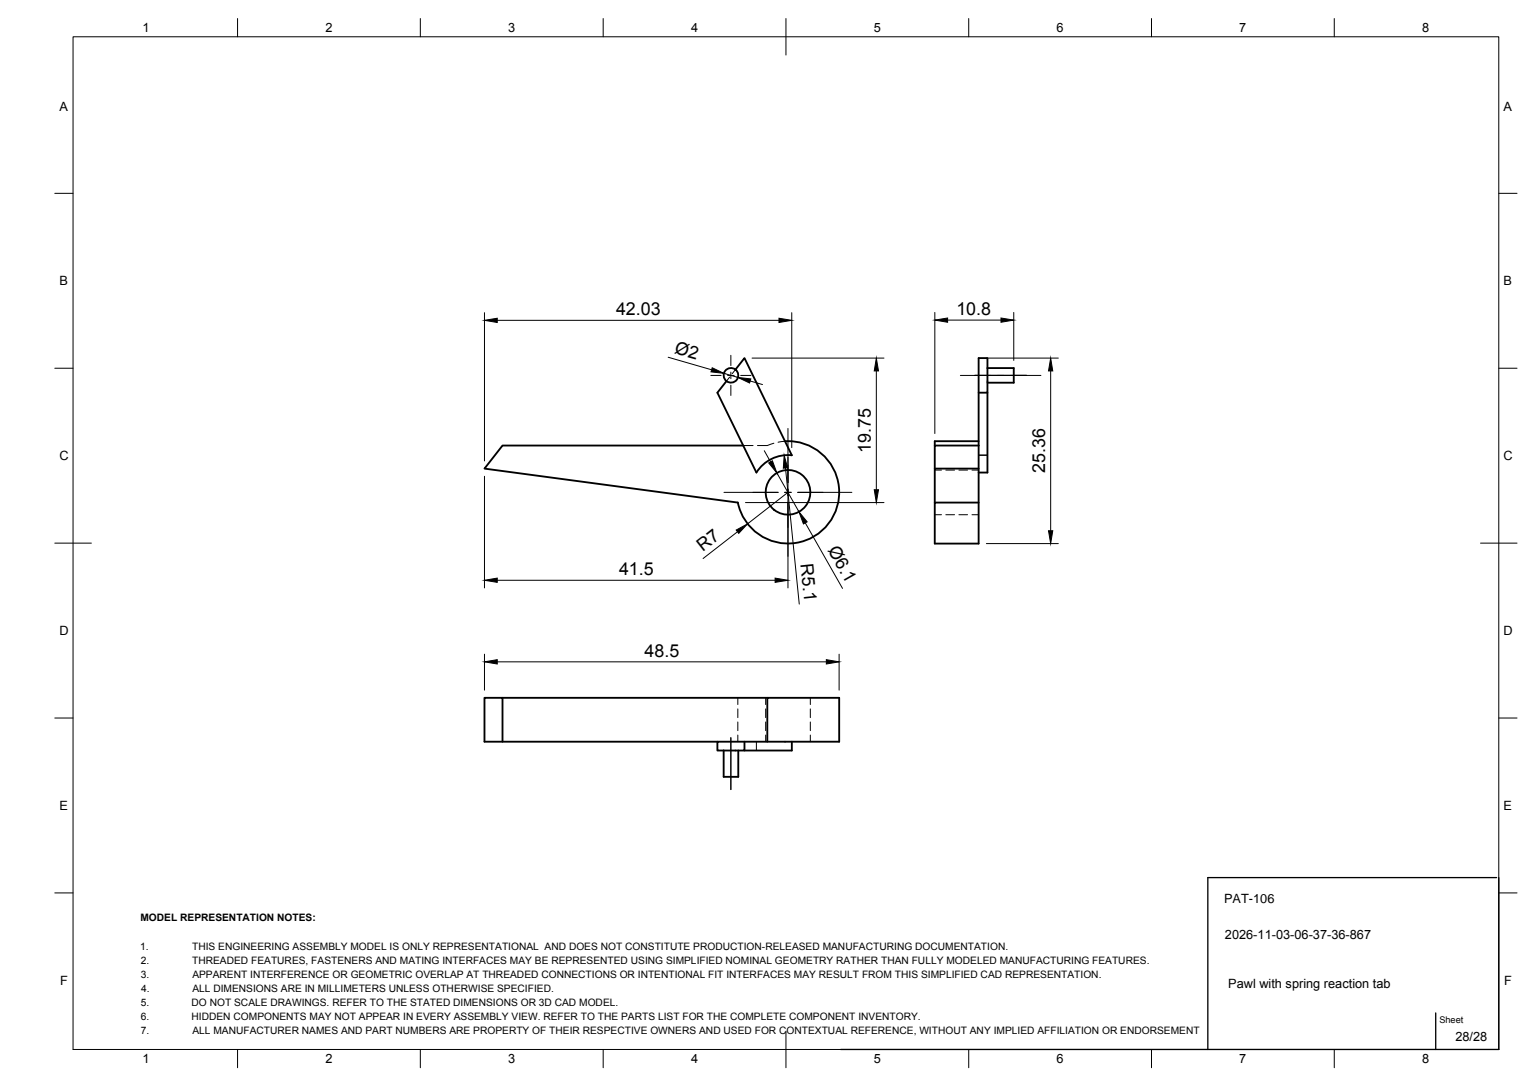
ISO-10303-21;
HEADER;
/* Generated by software containing ST-Developer
 * from STEP Tools, Inc. (www.steptools.com) 
 */

FILE_DESCRIPTION(
/* description */ ('Torsion-spring ratchet demonstrator'),
/* implementation_level */ '2;1');

FILE_NAME(
/* name */ 'Pawl with spring reaction tab.step',
/* time_stamp */ '2026-10-29T17:29:17-07:00',
/* author */ (''),
/* organization */ (''),
/* preprocessor_version */ 'ST-DEVELOPER v20.2',
/* originating_system */ 'Autodesk Translation Framework v15.17.0.0',
/* authorisation */ '');

FILE_SCHEMA (('AUTOMOTIVE_DESIGN { 1 0 10303 214 3 1 1 }'));
ENDSEC;

DATA;
#10=MECHANICAL_DESIGN_GEOMETRIC_PRESENTATION_REPRESENTATION('',(#314),#11258);
#258=SHAPE_REPRESENTATION_RELATIONSHIP('SRR','None',#11387,#282);
#282=ADVANCED_BREP_SHAPE_REPRESENTATION('',(#344),#11257);
#314=STYLED_ITEM('',(#11584),#344);
#344=MANIFOLD_SOLID_BREP('Body1',#5187);
#435=FACE_BOUND('',#1309,.T.);
#436=FACE_BOUND('',#1324,.T.);
#611=PLANE('',#6039);
#612=PLANE('',#6046);
#613=PLANE('',#6047);
#614=PLANE('',#6048);
#615=PLANE('',#6050);
#616=PLANE('',#6051);
#617=PLANE('',#6052);
#618=PLANE('',#6053);
#619=PLANE('',#6058);
#620=PLANE('',#6059);
#621=PLANE('',#6060);
#622=PLANE('',#6061);
#912=FACE_OUTER_BOUND('',#1307,.T.);
#913=FACE_OUTER_BOUND('',#1308,.T.);
#914=FACE_OUTER_BOUND('',#1310,.T.);
#915=FACE_OUTER_BOUND('',#1311,.T.);
#916=FACE_OUTER_BOUND('',#1312,.T.);
#917=FACE_OUTER_BOUND('',#1313,.T.);
#918=FACE_OUTER_BOUND('',#1314,.T.);
#919=FACE_OUTER_BOUND('',#1315,.T.);
#920=FACE_OUTER_BOUND('',#1316,.T.);
#921=FACE_OUTER_BOUND('',#1317,.T.);
#922=FACE_OUTER_BOUND('',#1318,.T.);
#923=FACE_OUTER_BOUND('',#1319,.T.);
#924=FACE_OUTER_BOUND('',#1320,.T.);
#925=FACE_OUTER_BOUND('',#1321,.T.);
#926=FACE_OUTER_BOUND('',#1322,.T.);
#927=FACE_OUTER_BOUND('',#1323,.T.);
#1307=EDGE_LOOP('',(#4690,#4691,#4692,#4693));
#1308=EDGE_LOOP('',(#4694,#4695,#4696,#4697,#4698,#4699,#4700));
#1309=EDGE_LOOP('',(#4701));
#1310=EDGE_LOOP('',(#4702,#4703,#4704,#4705,#4706));
#1311=EDGE_LOOP('',(#4707));
#1312=EDGE_LOOP('',(#4708,#4709));
#1313=EDGE_LOOP('',(#4710,#4711,#4712,#4713,#4714));
#1314=EDGE_LOOP('',(#4715,#4716,#4717,#4718,#4719,#4720));
#1315=EDGE_LOOP('',(#4721,#4722,#4723,#4724,#4725));
#1316=EDGE_LOOP('',(#4726,#4727,#4728,#4729,#4730));
#1317=EDGE_LOOP('',(#4731,#4732,#4733,#4734,#4735,#4736));
#1318=EDGE_LOOP('',(#4737,#4738,#4739,#4740));
#1319=EDGE_LOOP('',(#4741,#4742,#4743,#4744,#4745));
#1320=EDGE_LOOP('',(#4746,#4747,#4748,#4749));
#1321=EDGE_LOOP('',(#4750,#4751,#4752,#4753));
#1322=EDGE_LOOP('',(#4754,#4755,#4756,#4757,#4758));
#1323=EDGE_LOOP('',(#4759,#4760,#4761,#4762));
#1324=EDGE_LOOP('',(#4763));
#1681=LINE('',#11122,#2064);
#1682=LINE('',#11126,#2065);
#1683=LINE('',#11130,#2066);
#1684=LINE('',#11132,#2067);
#1685=LINE('',#11134,#2068);
#1686=LINE('',#11136,#2069);
#1687=LINE('',#11139,#2070);
#1688=LINE('',#11146,#2071);
#1689=LINE('',#11152,#2072);
#1690=LINE('',#11156,#2073);
#1691=LINE('',#11158,#2074);
#1692=LINE('',#11160,#2075);
#1693=LINE('',#11161,#2076);
#1694=LINE('',#11164,#2077);
#1695=LINE('',#11165,#2078);
#1696=LINE('',#11167,#2079);
#1697=LINE('',#11168,#2080);
#1698=LINE('',#11170,#2081);
#1699=LINE('',#11172,#2082);
#1700=LINE('',#11177,#2083);
#1701=LINE('',#11180,#2084);
#1702=LINE('',#11183,#2085);
#1703=LINE('',#11186,#2086);
#1704=LINE('',#11187,#2087);
#1705=LINE('',#11190,#2088);
#1706=LINE('',#11191,#2089);
#1707=LINE('',#11193,#2090);
#2064=VECTOR('',#7590,1.);
#2065=VECTOR('',#7593,1.);
#2066=VECTOR('',#7598,1.);
#2067=VECTOR('',#7599,1.);
#2068=VECTOR('',#7600,1.);
#2069=VECTOR('',#7601,1.);
#2070=VECTOR('',#7604,1.);
#2071=VECTOR('',#7611,0.0999999999999996);
#2072=VECTOR('',#7620,1.);
#2073=VECTOR('',#7625,1.);
#2074=VECTOR('',#7626,1.);
#2075=VECTOR('',#7627,1.);
#2076=VECTOR('',#7628,1.);
#2077=VECTOR('',#7631,1.);
#2078=VECTOR('',#7632,1.);
#2079=VECTOR('',#7633,1.);
#2080=VECTOR('',#7634,1.);
#2081=VECTOR('',#7637,1.);
#2082=VECTOR('',#7640,1.);
#2083=VECTOR('',#7647,0.305);
#2084=VECTOR('',#7650,1.);
#2085=VECTOR('',#7653,1.);
#2086=VECTOR('',#7656,1.);
#2087=VECTOR('',#7657,1.);
#2088=VECTOR('',#7660,1.);
#2089=VECTOR('',#7661,1.);
#2090=VECTOR('',#7664,1.);
#2325=CIRCLE('',#6037,0.51);
#2326=CIRCLE('',#6038,0.51);
#2327=CIRCLE('',#6040,0.7);
#2328=CIRCLE('',#6041,0.305);
#2329=CIRCLE('',#6043,0.0999999999999996);
#2330=CIRCLE('',#6044,0.0999999999999996);
#2331=CIRCLE('',#6045,0.0999999999999996);
#2332=CIRCLE('',#6049,0.7);
#2333=CIRCLE('',#6055,0.305);
#2334=CIRCLE('',#6057,0.7);
#2758=VERTEX_POINT('',#11120);
#2759=VERTEX_POINT('',#11121);
#2760=VERTEX_POINT('',#11123);
#2761=VERTEX_POINT('',#11125);
#2762=VERTEX_POINT('',#11129);
#2763=VERTEX_POINT('',#11131);
#2764=VERTEX_POINT('',#11133);
#2765=VERTEX_POINT('',#11135);
#2766=VERTEX_POINT('',#11137);
#2767=VERTEX_POINT('',#11140);
#2768=VERTEX_POINT('',#11143);
#2769=VERTEX_POINT('',#11145);
#2770=VERTEX_POINT('',#11147);
#2771=VERTEX_POINT('',#11154);
#2772=VERTEX_POINT('',#11157);
#2773=VERTEX_POINT('',#11159);
#2774=VERTEX_POINT('',#11163);
#2775=VERTEX_POINT('',#11166);
#2776=VERTEX_POINT('',#11175);
#2777=VERTEX_POINT('',#11179);
#2778=VERTEX_POINT('',#11181);
#2779=VERTEX_POINT('',#11185);
#2780=VERTEX_POINT('',#11189);
#3405=EDGE_CURVE('',#2758,#2759,#1681,.T.);
#3406=EDGE_CURVE('',#2760,#2758,#2325,.T.);
#3407=EDGE_CURVE('',#2761,#2760,#1682,.T.);
#3408=EDGE_CURVE('',#2759,#2761,#2326,.T.);
#3409=EDGE_CURVE('',#2761,#2762,#1683,.T.);
#3410=EDGE_CURVE('',#2762,#2763,#1684,.T.);
#3411=EDGE_CURVE('',#2763,#2764,#1685,.T.);
#3412=EDGE_CURVE('',#2764,#2765,#1686,.T.);
#3413=EDGE_CURVE('',#2765,#2766,#2327,.T.);
#3414=EDGE_CURVE('',#2766,#2759,#1687,.T.);
#3415=EDGE_CURVE('',#2767,#2767,#2328,.T.);
#3416=EDGE_CURVE('',#2768,#2768,#2329,.T.);
#3417=EDGE_CURVE('',#2768,#2769,#1688,.T.);
#3418=EDGE_CURVE('',#2770,#2769,#2330,.T.);
#3419=EDGE_CURVE('',#2770,#2769,#2331,.T.);
#3420=EDGE_CURVE('',#2770,#2769,#1689,.T.);
#3421=EDGE_CURVE('',#2766,#2771,#2332,.T.);
#3422=EDGE_CURVE('',#2771,#2762,#1690,.T.);
#3423=EDGE_CURVE('',#2772,#2762,#1691,.T.);
#3424=EDGE_CURVE('',#2773,#2772,#1692,.T.);
#3425=EDGE_CURVE('',#2766,#2773,#1693,.T.);
#3426=EDGE_CURVE('',#2772,#2774,#1694,.T.);
#3427=EDGE_CURVE('',#2769,#2774,#1695,.T.);
#3428=EDGE_CURVE('',#2775,#2770,#1696,.T.);
#3429=EDGE_CURVE('',#2773,#2775,#1697,.T.);
#3430=EDGE_CURVE('',#2758,#2775,#1698,.T.);
#3431=EDGE_CURVE('',#2774,#2760,#1699,.T.);
#3432=EDGE_CURVE('',#2776,#2776,#2333,.T.);
#3433=EDGE_CURVE('',#2776,#2767,#1700,.T.);
#3434=EDGE_CURVE('',#2777,#2765,#1701,.T.);
#3435=EDGE_CURVE('',#2777,#2778,#2334,.T.);
#3436=EDGE_CURVE('',#2771,#2778,#1702,.T.);
#3437=EDGE_CURVE('',#2779,#2764,#1703,.T.);
#3438=EDGE_CURVE('',#2777,#2779,#1704,.T.);
#3439=EDGE_CURVE('',#2779,#2780,#1705,.T.);
#3440=EDGE_CURVE('',#2780,#2763,#1706,.T.);
#3441=EDGE_CURVE('',#2780,#2778,#1707,.T.);
#4690=ORIENTED_EDGE('',*,*,#3405,.F.);
#4691=ORIENTED_EDGE('',*,*,#3406,.F.);
#4692=ORIENTED_EDGE('',*,*,#3407,.F.);
#4693=ORIENTED_EDGE('',*,*,#3408,.F.);
#4694=ORIENTED_EDGE('',*,*,#3408,.T.);
#4695=ORIENTED_EDGE('',*,*,#3409,.T.);
#4696=ORIENTED_EDGE('',*,*,#3410,.T.);
#4697=ORIENTED_EDGE('',*,*,#3411,.T.);
#4698=ORIENTED_EDGE('',*,*,#3412,.T.);
#4699=ORIENTED_EDGE('',*,*,#3413,.T.);
#4700=ORIENTED_EDGE('',*,*,#3414,.T.);
#4701=ORIENTED_EDGE('',*,*,#3415,.T.);
#4702=ORIENTED_EDGE('',*,*,#3416,.F.);
#4703=ORIENTED_EDGE('',*,*,#3417,.T.);
#4704=ORIENTED_EDGE('',*,*,#3418,.F.);
#4705=ORIENTED_EDGE('',*,*,#3419,.T.);
#4706=ORIENTED_EDGE('',*,*,#3417,.F.);
#4707=ORIENTED_EDGE('',*,*,#3416,.T.);
#4708=ORIENTED_EDGE('',*,*,#3420,.T.);
#4709=ORIENTED_EDGE('',*,*,#3419,.F.);
#4710=ORIENTED_EDGE('',*,*,#3421,.T.);
#4711=ORIENTED_EDGE('',*,*,#3422,.T.);
#4712=ORIENTED_EDGE('',*,*,#3423,.F.);
#4713=ORIENTED_EDGE('',*,*,#3424,.F.);
#4714=ORIENTED_EDGE('',*,*,#3425,.F.);
#4715=ORIENTED_EDGE('',*,*,#3424,.T.);
#4716=ORIENTED_EDGE('',*,*,#3426,.T.);
#4717=ORIENTED_EDGE('',*,*,#3427,.F.);
#4718=ORIENTED_EDGE('',*,*,#3420,.F.);
#4719=ORIENTED_EDGE('',*,*,#3428,.F.);
#4720=ORIENTED_EDGE('',*,*,#3429,.F.);
#4721=ORIENTED_EDGE('',*,*,#3405,.T.);
#4722=ORIENTED_EDGE('',*,*,#3414,.F.);
#4723=ORIENTED_EDGE('',*,*,#3425,.T.);
#4724=ORIENTED_EDGE('',*,*,#3429,.T.);
#4725=ORIENTED_EDGE('',*,*,#3430,.F.);
#4726=ORIENTED_EDGE('',*,*,#3407,.T.);
#4727=ORIENTED_EDGE('',*,*,#3431,.F.);
#4728=ORIENTED_EDGE('',*,*,#3426,.F.);
#4729=ORIENTED_EDGE('',*,*,#3423,.T.);
#4730=ORIENTED_EDGE('',*,*,#3409,.F.);
#4731=ORIENTED_EDGE('',*,*,#3406,.T.);
#4732=ORIENTED_EDGE('',*,*,#3430,.T.);
#4733=ORIENTED_EDGE('',*,*,#3428,.T.);
#4734=ORIENTED_EDGE('',*,*,#3418,.T.);
#4735=ORIENTED_EDGE('',*,*,#3427,.T.);
#4736=ORIENTED_EDGE('',*,*,#3431,.T.);
#4737=ORIENTED_EDGE('',*,*,#3432,.F.);
#4738=ORIENTED_EDGE('',*,*,#3433,.T.);
#4739=ORIENTED_EDGE('',*,*,#3415,.F.);
#4740=ORIENTED_EDGE('',*,*,#3433,.F.);
#4741=ORIENTED_EDGE('',*,*,#3434,.F.);
#4742=ORIENTED_EDGE('',*,*,#3435,.T.);
#4743=ORIENTED_EDGE('',*,*,#3436,.F.);
#4744=ORIENTED_EDGE('',*,*,#3421,.F.);
#4745=ORIENTED_EDGE('',*,*,#3413,.F.);
#4746=ORIENTED_EDGE('',*,*,#3434,.T.);
#4747=ORIENTED_EDGE('',*,*,#3412,.F.);
#4748=ORIENTED_EDGE('',*,*,#3437,.F.);
#4749=ORIENTED_EDGE('',*,*,#3438,.F.);
#4750=ORIENTED_EDGE('',*,*,#3439,.F.);
#4751=ORIENTED_EDGE('',*,*,#3437,.T.);
#4752=ORIENTED_EDGE('',*,*,#3411,.F.);
#4753=ORIENTED_EDGE('',*,*,#3440,.F.);
#4754=ORIENTED_EDGE('',*,*,#3436,.T.);
#4755=ORIENTED_EDGE('',*,*,#3441,.F.);
#4756=ORIENTED_EDGE('',*,*,#3440,.T.);
#4757=ORIENTED_EDGE('',*,*,#3410,.F.);
#4758=ORIENTED_EDGE('',*,*,#3422,.F.);
#4759=ORIENTED_EDGE('',*,*,#3438,.T.);
#4760=ORIENTED_EDGE('',*,*,#3439,.T.);
#4761=ORIENTED_EDGE('',*,*,#3441,.T.);
#4762=ORIENTED_EDGE('',*,*,#3435,.F.);
#4763=ORIENTED_EDGE('',*,*,#3432,.T.);
#4845=CYLINDRICAL_SURFACE('',#6036,0.51);
#4846=CYLINDRICAL_SURFACE('',#6042,0.0999999999999996);
#4847=CYLINDRICAL_SURFACE('',#6054,0.305);
#4848=CYLINDRICAL_SURFACE('',#6056,0.7);
#5138=ADVANCED_FACE('',(#912),#4845,.F.);
#5139=ADVANCED_FACE('',(#913,#435),#611,.T.);
#5140=ADVANCED_FACE('',(#914),#4846,.T.);
#5141=ADVANCED_FACE('',(#915),#612,.T.);
#5142=ADVANCED_FACE('',(#916),#613,.F.);
#5143=ADVANCED_FACE('',(#917),#614,.F.);
#5144=ADVANCED_FACE('',(#918),#615,.T.);
#5145=ADVANCED_FACE('',(#919),#616,.T.);
#5146=ADVANCED_FACE('',(#920),#617,.T.);
#5147=ADVANCED_FACE('',(#921),#618,.T.);
#5148=ADVANCED_FACE('',(#922),#4847,.F.);
#5149=ADVANCED_FACE('',(#923),#4848,.T.);
#5150=ADVANCED_FACE('',(#924),#619,.T.);
#5151=ADVANCED_FACE('',(#925),#620,.T.);
#5152=ADVANCED_FACE('',(#926),#621,.T.);
#5153=ADVANCED_FACE('',(#927,#436),#622,.F.);
#5187=CLOSED_SHELL('',(#5138,#5139,#5140,#5141,#5142,#5143,#5144,#5145,
#5146,#5147,#5148,#5149,#5150,#5151,#5152,#5153));
#6035=AXIS2_PLACEMENT_3D('',#11118,#7586,#7587);
#6036=AXIS2_PLACEMENT_3D('',#11119,#7588,#7589);
#6037=AXIS2_PLACEMENT_3D('',#11124,#7591,#7592);
#6038=AXIS2_PLACEMENT_3D('',#11127,#7594,#7595);
#6039=AXIS2_PLACEMENT_3D('',#11128,#7596,#7597);
#6040=AXIS2_PLACEMENT_3D('',#11138,#7602,#7603);
#6041=AXIS2_PLACEMENT_3D('',#11141,#7605,#7606);
#6042=AXIS2_PLACEMENT_3D('',#11142,#7607,#7608);
#6043=AXIS2_PLACEMENT_3D('',#11144,#7609,#7610);
#6044=AXIS2_PLACEMENT_3D('',#11148,#7612,#7613);
#6045=AXIS2_PLACEMENT_3D('',#11149,#7614,#7615);
#6046=AXIS2_PLACEMENT_3D('',#11150,#7616,#7617);
#6047=AXIS2_PLACEMENT_3D('',#11151,#7618,#7619);
#6048=AXIS2_PLACEMENT_3D('',#11153,#7621,#7622);
#6049=AXIS2_PLACEMENT_3D('',#11155,#7623,#7624);
#6050=AXIS2_PLACEMENT_3D('',#11162,#7629,#7630);
#6051=AXIS2_PLACEMENT_3D('',#11169,#7635,#7636);
#6052=AXIS2_PLACEMENT_3D('',#11171,#7638,#7639);
#6053=AXIS2_PLACEMENT_3D('',#11173,#7641,#7642);
#6054=AXIS2_PLACEMENT_3D('',#11174,#7643,#7644);
#6055=AXIS2_PLACEMENT_3D('',#11176,#7645,#7646);
#6056=AXIS2_PLACEMENT_3D('',#11178,#7648,#7649);
#6057=AXIS2_PLACEMENT_3D('',#11182,#7651,#7652);
#6058=AXIS2_PLACEMENT_3D('',#11184,#7654,#7655);
#6059=AXIS2_PLACEMENT_3D('',#11188,#7658,#7659);
#6060=AXIS2_PLACEMENT_3D('',#11192,#7662,#7663);
#6061=AXIS2_PLACEMENT_3D('',#11194,#7665,#7666);
#7586=DIRECTION('axis',(0.,0.,1.));
#7587=DIRECTION('refdir',(1.,0.,0.));
#7588=DIRECTION('center_axis',(0.,0.,1.));
#7589=DIRECTION('ref_axis',(1.,0.,0.));
#7590=DIRECTION('',(0.,0.,-1.));
#7591=DIRECTION('center_axis',(0.,0.,-1.));
#7592=DIRECTION('ref_axis',(1.,0.,0.));
#7593=DIRECTION('',(0.,0.,1.));
#7594=DIRECTION('center_axis',(0.,0.,1.));
#7595=DIRECTION('ref_axis',(1.,0.,0.));
#7596=DIRECTION('center_axis',(0.,2.22044604925031E-16,1.));
#7597=DIRECTION('ref_axis',(0.,-1.,2.22044604925031E-16));
#7598=DIRECTION('',(0.438202247191011,0.898876404494382,-1.99590656112388E-16));
#7599=DIRECTION('',(-0.615893007805892,0.78782980581837,-1.74933357981104E-16));
#7600=DIRECTION('',(-1.,0.,0.));
#7601=DIRECTION('',(0.50579161179386,-0.862655693448417,1.91548042638083E-16));
#7602=DIRECTION('center_axis',(0.,2.22044604925031E-16,1.));
#7603=DIRECTION('ref_axis',(1.,0.,0.));
#7604=DIRECTION('',(-0.438202247191011,-0.898876404494382,1.99590656112388E-16));
#7605=DIRECTION('center_axis',(0.,-2.22044604925031E-16,-1.));
#7606=DIRECTION('ref_axis',(1.,0.,0.));
#7607=DIRECTION('center_axis',(0.,0.,1.));
#7608=DIRECTION('ref_axis',(1.,0.,0.));
#7609=DIRECTION('center_axis',(0.,0.,1.));
#7610=DIRECTION('ref_axis',(1.,0.,0.));
#7611=DIRECTION('',(0.,0.,-1.));
#7612=DIRECTION('center_axis',(0.,0.,-1.));
#7613=DIRECTION('ref_axis',(1.,0.,0.));
#7614=DIRECTION('center_axis',(0.,0.,1.));
#7615=DIRECTION('ref_axis',(1.,0.,0.));
#7616=DIRECTION('center_axis',(0.,0.,1.));
#7617=DIRECTION('ref_axis',(1.,0.,0.));
#7618=DIRECTION('center_axis',(0.,0.,1.));
#7619=DIRECTION('ref_axis',(1.,0.,0.));
#7620=DIRECTION('',(-1.,0.,0.));
#7621=DIRECTION('center_axis',(0.,0.,1.));
#7622=DIRECTION('ref_axis',(1.,0.,0.));
#7623=DIRECTION('center_axis',(0.,2.22044604925031E-16,1.));
#7624=DIRECTION('ref_axis',(1.,0.,0.));
#7625=DIRECTION('',(-0.615893007805892,0.78782980581837,-1.74933357981104E-16));
#7626=DIRECTION('',(-0.438202247191011,-0.898876404494382,0.));
#7627=DIRECTION('',(-1.,0.,0.));
#7628=DIRECTION('',(0.438202247191011,0.898876404494382,0.));
#7629=DIRECTION('center_axis',(0.,1.,0.));
#7630=DIRECTION('ref_axis',(-1.,0.,0.));
#7631=DIRECTION('',(0.,0.,1.));
#7632=DIRECTION('',(-1.,0.,0.));
#7633=DIRECTION('',(-1.,0.,0.));
#7634=DIRECTION('',(0.,0.,1.));
#7635=DIRECTION('center_axis',(0.898876404494382,-0.438202247191011,0.));
#7636=DIRECTION('ref_axis',(0.438202247191011,0.898876404494382,0.));
#7637=DIRECTION('',(0.438202247191011,0.898876404494382,0.));
#7638=DIRECTION('center_axis',(-0.898876404494382,0.438202247191011,0.));
#7639=DIRECTION('ref_axis',(-0.438202247191011,-0.898876404494382,0.));
#7640=DIRECTION('',(-0.438202247191011,-0.898876404494382,0.));
#7641=DIRECTION('center_axis',(0.,0.,1.));
#7642=DIRECTION('ref_axis',(1.,0.,0.));
#7643=DIRECTION('center_axis',(0.,2.22044604925031E-16,1.));
#7644=DIRECTION('ref_axis',(1.,0.,0.));
#7645=DIRECTION('center_axis',(0.,2.22044604925031E-16,1.));
#7646=DIRECTION('ref_axis',(1.,0.,0.));
#7647=DIRECTION('',(0.,2.22044604925031E-16,1.));
#7648=DIRECTION('center_axis',(0.,2.22044604925031E-16,1.));
#7649=DIRECTION('ref_axis',(0.185131832090925,-0.982713694189034,2.18206273980622E-16));
#7650=DIRECTION('',(0.,2.22044604925031E-16,1.));
#7651=DIRECTION('center_axis',(0.,2.22044604925031E-16,1.));
#7652=DIRECTION('ref_axis',(1.,0.,0.));
#7653=DIRECTION('',(0.,-2.22044604925031E-16,-1.));
#7654=DIRECTION('center_axis',(-0.862655693448417,-0.50579161179386,1.12308298615162E-16));
#7655=DIRECTION('ref_axis',(0.50579161179386,-0.862655693448417,1.91548042638083E-16));
#7656=DIRECTION('',(0.,2.22044604925031E-16,1.));
#7657=DIRECTION('',(-0.50579161179386,0.862655693448417,-1.91548042638083E-16));
#7658=DIRECTION('center_axis',(0.,1.,-2.22044604925031E-16));
#7659=DIRECTION('ref_axis',(-1.,0.,0.));
#7660=DIRECTION('',(1.,0.,0.));
#7661=DIRECTION('',(0.,2.22044604925031E-16,1.));
#7662=DIRECTION('center_axis',(0.78782980581837,0.615893007805892,-1.36755719594349E-16));
#7663=DIRECTION('ref_axis',(-0.615893007805892,0.78782980581837,-1.74933357981104E-16));
#7664=DIRECTION('',(0.615893007805892,-0.78782980581837,1.74933357981104E-16));
#7665=DIRECTION('center_axis',(0.,2.22044604925031E-16,1.));
#7666=DIRECTION('ref_axis',(1.,0.,0.));
#11118=CARTESIAN_POINT('',(0.,0.,0.));
#11119=CARTESIAN_POINT('Origin',(6.5,-3.47,5.4));
#11120=CARTESIAN_POINT('',(6.93208101356604,-3.19906458755684,5.52));
#11121=CARTESIAN_POINT('',(6.93208101356604,-3.19906458755684,5.4));
#11122=CARTESIAN_POINT('',(6.93208101356604,-3.19906458755684,5.4));
#11123=CARTESIAN_POINT('',(6.44729373923199,-2.96273079131899,5.52));
#11124=CARTESIAN_POINT('Origin',(6.5,-3.47,5.52));
#11125=CARTESIAN_POINT('',(6.44729373923199,-2.96273079131899,5.4));
#11126=CARTESIAN_POINT('',(6.44729373923199,-2.96273079131899,5.4));
#11127=CARTESIAN_POINT('Origin',(6.5,-3.47,5.4));
#11128=CARTESIAN_POINT('Origin',(5.6,-1.935,5.4));
#11129=CARTESIAN_POINT('',(6.627369839284,-2.59334391941745,5.4));
#11130=CARTESIAN_POINT('',(6.83470395152127,-2.16804317636662,5.4));
#11131=CARTESIAN_POINT('',(4.6,-8.88178419700125E-16,5.4));
#11132=CARTESIAN_POINT('',(4.6,-8.88178419700125E-16,5.4));
#11133=CARTESIAN_POINT('',(4.2,-8.88178419700125E-16,5.4));
#11134=CARTESIAN_POINT('',(4.2,-8.88178419700125E-16,5.4));
#11135=CARTESIAN_POINT('',(5.96787188180707,-3.01520370952651,5.4));
#11136=CARTESIAN_POINT('',(6.,-3.07,5.4));
#11137=CARTESIAN_POINT('',(7.02546072606318,-3.00751645935757,5.4));
#11138=CARTESIAN_POINT('Origin',(6.5,-3.47,5.4));
#11139=CARTESIAN_POINT('',(6.9870975886883,-3.08621007448555,5.4));
#11140=CARTESIAN_POINT('',(6.195,-3.47,5.4));
#11141=CARTESIAN_POINT('Origin',(6.5,-3.47,5.4));
#11142=CARTESIAN_POINT('Origin',(7.28,-1.87,5.52));
#11143=CARTESIAN_POINT('',(7.18,-1.87,5.88));
#11144=CARTESIAN_POINT('Origin',(7.28,-1.87,5.88));
#11145=CARTESIAN_POINT('',(7.18,-1.87,5.52));
#11146=CARTESIAN_POINT('',(7.18,-1.87,5.52));
#11147=CARTESIAN_POINT('',(7.38,-1.87,5.52));
#11148=CARTESIAN_POINT('Origin',(7.28,-1.87,5.52));
#11149=CARTESIAN_POINT('Origin',(7.28,-1.87,5.52));
#11150=CARTESIAN_POINT('Origin',(7.28,-1.87,5.88));
#11151=CARTESIAN_POINT('Origin',(7.28,-1.87,5.52));
#11152=CARTESIAN_POINT('',(7.58,-1.87,5.52));
#11153=CARTESIAN_POINT('Origin',(6.89,-2.67,5.4));
#11154=CARTESIAN_POINT('',(6.83016839641497,-2.85275707374749,5.4));
#11155=CARTESIAN_POINT('Origin',(6.5,-3.47,5.4));
#11156=CARTESIAN_POINT('',(4.6,-8.88178419700125E-16,5.4));
#11157=CARTESIAN_POINT('',(6.98,-1.87,5.4));
#11158=CARTESIAN_POINT('',(6.98,-1.87,5.4));
#11159=CARTESIAN_POINT('',(7.58,-1.87,5.4));
#11160=CARTESIAN_POINT('',(7.58,-1.87,5.4));
#11161=CARTESIAN_POINT('',(6.8,-3.47,5.4));
#11162=CARTESIAN_POINT('Origin',(7.58,-1.87,5.4));
#11163=CARTESIAN_POINT('',(6.98,-1.87,5.52));
#11164=CARTESIAN_POINT('',(6.98,-1.87,5.4));
#11165=CARTESIAN_POINT('',(7.58,-1.87,5.52));
#11166=CARTESIAN_POINT('',(7.58,-1.87,5.52));
#11167=CARTESIAN_POINT('',(7.58,-1.87,5.52));
#11168=CARTESIAN_POINT('',(7.58,-1.87,5.4));
#11169=CARTESIAN_POINT('Origin',(6.8,-3.47,5.4));
#11170=CARTESIAN_POINT('',(6.8,-3.47,5.52));
#11171=CARTESIAN_POINT('Origin',(6.98,-1.87,5.4));
#11172=CARTESIAN_POINT('',(6.98,-1.87,5.52));
#11173=CARTESIAN_POINT('Origin',(6.89,-2.67,5.52));
#11174=CARTESIAN_POINT('Origin',(6.5,-3.47,4.7));
#11175=CARTESIAN_POINT('',(6.195,-3.47,4.8));
#11176=CARTESIAN_POINT('Origin',(6.5,-3.47,4.8));
#11177=CARTESIAN_POINT('',(6.195,-3.47,4.7));
#11178=CARTESIAN_POINT('Origin',(6.5,-3.47,4.8));
#11179=CARTESIAN_POINT('',(5.96787188180707,-3.01520370952651,4.8));
#11180=CARTESIAN_POINT('',(5.96787188180707,-3.01520370952651,4.8));
#11181=CARTESIAN_POINT('',(6.83016839641497,-2.85275707374749,4.8));
#11182=CARTESIAN_POINT('Origin',(6.5,-3.47,4.8));
#11183=CARTESIAN_POINT('',(6.83016839641497,-2.85275707374749,4.8));
#11184=CARTESIAN_POINT('Origin',(4.2,-8.88178419700125E-16,4.8));
#11185=CARTESIAN_POINT('',(4.2,-8.88178419700125E-16,4.8));
#11186=CARTESIAN_POINT('',(4.2,-8.88178419700125E-16,4.8));
#11187=CARTESIAN_POINT('',(6.,-3.07,4.8));
#11188=CARTESIAN_POINT('Origin',(4.6,-8.88178419700125E-16,4.8));
#11189=CARTESIAN_POINT('',(4.6,-8.88178419700125E-16,4.8));
#11190=CARTESIAN_POINT('',(4.2,-8.88178419700125E-16,4.8));
#11191=CARTESIAN_POINT('',(4.6,-8.88178419700125E-16,4.8));
#11192=CARTESIAN_POINT('Origin',(7.,-3.07,4.8));
#11193=CARTESIAN_POINT('',(4.6,-8.88178419700125E-16,4.8));
#11194=CARTESIAN_POINT('Origin',(5.6,-1.935,4.8));
#11227=UNCERTAINTY_MEASURE_WITH_UNIT(LENGTH_MEASURE(0.001),#11259,
'DISTANCE_ACCURACY_VALUE',
'Maximum model space distance between geometric entities at asserted c
onnectivities');
#11228=UNCERTAINTY_MEASURE_WITH_UNIT(LENGTH_MEASURE(0.001),#11259,
'DISTANCE_ACCURACY_VALUE',
'Maximum model space distance between geometric entities at asserted c
onnectivities');
#11257=(
GEOMETRIC_REPRESENTATION_CONTEXT(3)
GLOBAL_UNCERTAINTY_ASSIGNED_CONTEXT((#11227))
GLOBAL_UNIT_ASSIGNED_CONTEXT((#11259,#11261,#11262))
REPRESENTATION_CONTEXT('','3D')
);
#11258=(
GEOMETRIC_REPRESENTATION_CONTEXT(3)
GLOBAL_UNCERTAINTY_ASSIGNED_CONTEXT((#11228))
GLOBAL_UNIT_ASSIGNED_CONTEXT((#11259,#11261,#11262))
REPRESENTATION_CONTEXT('','3D')
);
#11259=(
LENGTH_UNIT()
NAMED_UNIT(*)
SI_UNIT(.CENTI.,.METRE.)
);
#11261=(
NAMED_UNIT(*)
PLANE_ANGLE_UNIT()
SI_UNIT($,.RADIAN.)
);
#11262=(
NAMED_UNIT(*)
SI_UNIT($,.STERADIAN.)
SOLID_ANGLE_UNIT()
);
#11291=SHAPE_DEFINITION_REPRESENTATION(#11354,#11387);
#11354=PRODUCT_DEFINITION_SHAPE('',$,#11417);
#11387=SHAPE_REPRESENTATION('',(#6035),#11257);
#11388=PRODUCT_DEFINITION_CONTEXT('part definition',#11477,'design');
#11417=PRODUCT_DEFINITION('Pawl with spring reaction tab',
'Pawl with spring reaction tab',#11446,#11388);
#11446=PRODUCT_DEFINITION_FORMATION('',$,#11507);
#11477=APPLICATION_CONTEXT(
'Core Data for Automotive Mechanical Design Process');
#11478=PRODUCT_CONTEXT('part definition',#11477,'mechanical');
#11507=PRODUCT('Pawl with spring reaction tab',
'Pawl with spring reaction tab','Pawl with spring reaction tab',(#11478));
#11578=COLOUR_RGB('Grey',0.48,0.52,0.57);
#11579=FILL_AREA_STYLE_COLOUR('',#11578);
#11580=FILL_AREA_STYLE('',(#11579));
#11581=SURFACE_STYLE_FILL_AREA(#11580);
#11582=SURFACE_SIDE_STYLE('',(#11581));
#11583=SURFACE_STYLE_USAGE(.BOTH.,#11582);
#11584=PRESENTATION_STYLE_ASSIGNMENT((#11583));
ENDSEC;
END-ISO-10303-21;
